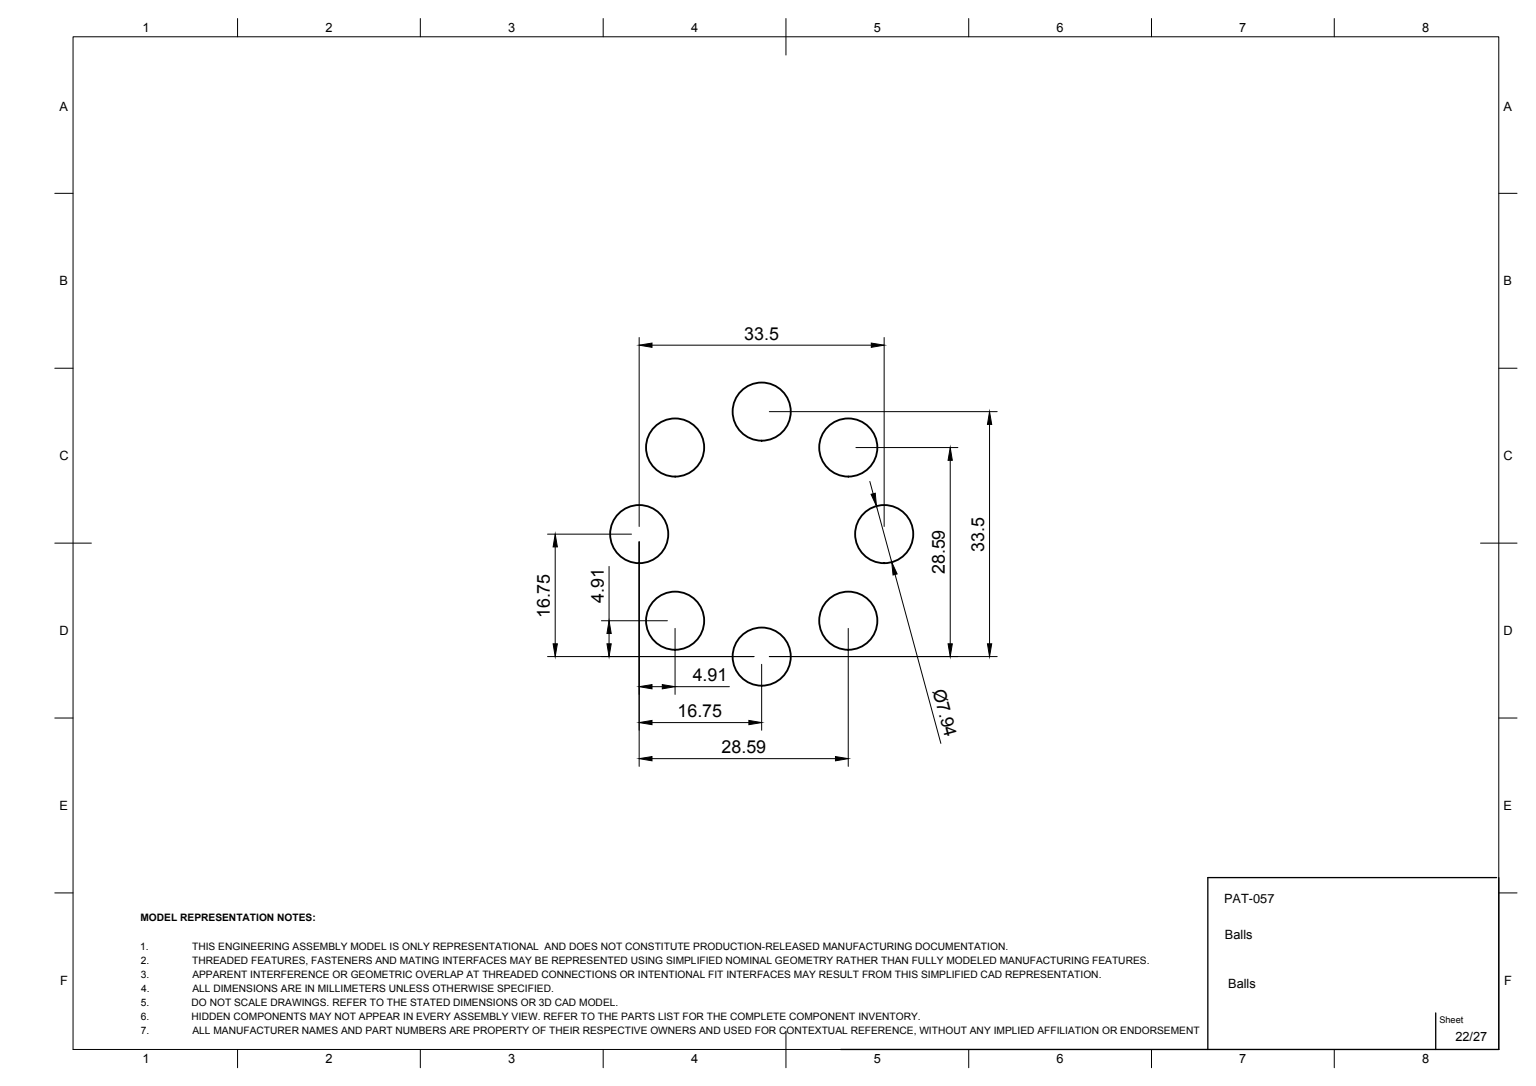
ISO-10303-21;
HEADER;
/* Generated by software containing ST-Developer
 * from STEP Tools, Inc. (www.steptools.com) 
 */

FILE_DESCRIPTION(
/* description */ ('Bearing-mounted hook block'),
/* implementation_level */ '2;1');

FILE_NAME(
/* name */ 'Balls.step',
/* time_stamp */ '2026-10-28T22:30:11-07:00',
/* author */ (''),
/* organization */ (''),
/* preprocessor_version */ 'ST-DEVELOPER v20.2',
/* originating_system */ 'Autodesk Translation Framework v15.17.0.0',
/* authorisation */ '');

FILE_SCHEMA (('AUTOMOTIVE_DESIGN { 1 0 10303 214 3 1 1 }'));
ENDSEC;

DATA;
#10=MECHANICAL_DESIGN_GEOMETRIC_PRESENTATION_REPRESENTATION('',(#339,#340,#341,#342,#343,#344,#345,#346),#7609);
#29=SPHERICAL_SURFACE('',#4545,0.3969);
#30=SPHERICAL_SURFACE('',#4547,0.3969);
#31=SPHERICAL_SURFACE('',#4549,0.3969);
#32=SPHERICAL_SURFACE('',#4551,0.3969);
#33=SPHERICAL_SURFACE('',#4553,0.3969);
#34=SPHERICAL_SURFACE('',#4555,0.3969);
#35=SPHERICAL_SURFACE('',#4557,0.3969);
#36=SPHERICAL_SURFACE('',#4559,0.3969);
#291=SHAPE_REPRESENTATION_RELATIONSHIP('SRR','None',#7740,#315);
#315=ADVANCED_BREP_SHAPE_REPRESENTATION('',(#369,#370,#371,#372,#373,#374,
#375,#376),#7600);
#339=STYLED_ITEM('',(#7931),#369);
#340=STYLED_ITEM('',(#7931),#370);
#341=STYLED_ITEM('',(#7931),#371);
#342=STYLED_ITEM('',(#7931),#372);
#343=STYLED_ITEM('',(#7931),#373);
#344=STYLED_ITEM('',(#7931),#374);
#345=STYLED_ITEM('',(#7931),#375);
#346=STYLED_ITEM('',(#7931),#376);
#369=MANIFOLD_SOLID_BREP('Body1',#3937);
#370=MANIFOLD_SOLID_BREP('Body2',#3938);
#371=MANIFOLD_SOLID_BREP('Body3',#3939);
#372=MANIFOLD_SOLID_BREP('Body4',#3940);
#373=MANIFOLD_SOLID_BREP('Body5',#3941);
#374=MANIFOLD_SOLID_BREP('Body6',#3942);
#375=MANIFOLD_SOLID_BREP('Body7',#3943);
#376=MANIFOLD_SOLID_BREP('Body8',#3944);
#1147=FACE_OUTER_BOUND('',#1440,.T.);
#1148=FACE_OUTER_BOUND('',#1441,.T.);
#1149=FACE_OUTER_BOUND('',#1442,.T.);
#1150=FACE_OUTER_BOUND('',#1443,.T.);
#1151=FACE_OUTER_BOUND('',#1444,.T.);
#1152=FACE_OUTER_BOUND('',#1445,.T.);
#1153=FACE_OUTER_BOUND('',#1446,.T.);
#1154=FACE_OUTER_BOUND('',#1447,.T.);
#1440=EDGE_LOOP('',(#3188,#3189));
#1441=EDGE_LOOP('',(#3190,#3191));
#1442=EDGE_LOOP('',(#3192,#3193));
#1443=EDGE_LOOP('',(#3194,#3195));
#1444=EDGE_LOOP('',(#3196,#3197));
#1445=EDGE_LOOP('',(#3198,#3199));
#1446=EDGE_LOOP('',(#3200,#3201));
#1447=EDGE_LOOP('',(#3202,#3203));
#1689=CIRCLE('',#4546,0.3969);
#1690=CIRCLE('',#4548,0.3969);
#1691=CIRCLE('',#4550,0.3969);
#1692=CIRCLE('',#4552,0.3969);
#1693=CIRCLE('',#4554,0.3969);
#1694=CIRCLE('',#4556,0.3969);
#1695=CIRCLE('',#4558,0.3969);
#1696=CIRCLE('',#4560,0.3969);
#1972=VERTEX_POINT('',#6771);
#1973=VERTEX_POINT('',#6772);
#1974=VERTEX_POINT('',#6775);
#1975=VERTEX_POINT('',#6776);
#1976=VERTEX_POINT('',#6779);
#1977=VERTEX_POINT('',#6780);
#1978=VERTEX_POINT('',#6783);
#1979=VERTEX_POINT('',#6784);
#1980=VERTEX_POINT('',#6787);
#1981=VERTEX_POINT('',#6788);
#1982=VERTEX_POINT('',#6791);
#1983=VERTEX_POINT('',#6792);
#1984=VERTEX_POINT('',#6795);
#1985=VERTEX_POINT('',#6796);
#1986=VERTEX_POINT('',#6799);
#1987=VERTEX_POINT('',#6800);
#2404=EDGE_CURVE('',#1972,#1973,#1689,.T.);
#2405=EDGE_CURVE('',#1974,#1975,#1690,.T.);
#2406=EDGE_CURVE('',#1976,#1977,#1691,.T.);
#2407=EDGE_CURVE('',#1978,#1979,#1692,.T.);
#2408=EDGE_CURVE('',#1980,#1981,#1693,.T.);
#2409=EDGE_CURVE('',#1982,#1983,#1694,.T.);
#2410=EDGE_CURVE('',#1984,#1985,#1695,.T.);
#2411=EDGE_CURVE('',#1986,#1987,#1696,.T.);
#3188=ORIENTED_EDGE('',*,*,#2404,.T.);
#3189=ORIENTED_EDGE('',*,*,#2404,.F.);
#3190=ORIENTED_EDGE('',*,*,#2405,.T.);
#3191=ORIENTED_EDGE('',*,*,#2405,.F.);
#3192=ORIENTED_EDGE('',*,*,#2406,.T.);
#3193=ORIENTED_EDGE('',*,*,#2406,.F.);
#3194=ORIENTED_EDGE('',*,*,#2407,.T.);
#3195=ORIENTED_EDGE('',*,*,#2407,.F.);
#3196=ORIENTED_EDGE('',*,*,#2408,.T.);
#3197=ORIENTED_EDGE('',*,*,#2408,.F.);
#3198=ORIENTED_EDGE('',*,*,#2409,.T.);
#3199=ORIENTED_EDGE('',*,*,#2409,.F.);
#3200=ORIENTED_EDGE('',*,*,#2410,.T.);
#3201=ORIENTED_EDGE('',*,*,#2410,.F.);
#3202=ORIENTED_EDGE('',*,*,#2411,.T.);
#3203=ORIENTED_EDGE('',*,*,#2411,.F.);
#3829=ADVANCED_FACE('',(#1147),#29,.T.);
#3830=ADVANCED_FACE('',(#1148),#30,.T.);
#3831=ADVANCED_FACE('',(#1149),#31,.T.);
#3832=ADVANCED_FACE('',(#1150),#32,.T.);
#3833=ADVANCED_FACE('',(#1151),#33,.T.);
#3834=ADVANCED_FACE('',(#1152),#34,.T.);
#3835=ADVANCED_FACE('',(#1153),#35,.T.);
#3836=ADVANCED_FACE('',(#1154),#36,.T.);
#3937=CLOSED_SHELL('',(#3829));
#3938=CLOSED_SHELL('',(#3830));
#3939=CLOSED_SHELL('',(#3831));
#3940=CLOSED_SHELL('',(#3832));
#3941=CLOSED_SHELL('',(#3833));
#3942=CLOSED_SHELL('',(#3834));
#3943=CLOSED_SHELL('',(#3835));
#3944=CLOSED_SHELL('',(#3836));
#4544=AXIS2_PLACEMENT_3D('',#6769,#5558,#5559);
#4545=AXIS2_PLACEMENT_3D('',#6770,#5560,#5561);
#4546=AXIS2_PLACEMENT_3D('',#6773,#5562,#5563);
#4547=AXIS2_PLACEMENT_3D('',#6774,#5564,#5565);
#4548=AXIS2_PLACEMENT_3D('',#6777,#5566,#5567);
#4549=AXIS2_PLACEMENT_3D('',#6778,#5568,#5569);
#4550=AXIS2_PLACEMENT_3D('',#6781,#5570,#5571);
#4551=AXIS2_PLACEMENT_3D('',#6782,#5572,#5573);
#4552=AXIS2_PLACEMENT_3D('',#6785,#5574,#5575);
#4553=AXIS2_PLACEMENT_3D('',#6786,#5576,#5577);
#4554=AXIS2_PLACEMENT_3D('',#6789,#5578,#5579);
#4555=AXIS2_PLACEMENT_3D('',#6790,#5580,#5581);
#4556=AXIS2_PLACEMENT_3D('',#6793,#5582,#5583);
#4557=AXIS2_PLACEMENT_3D('',#6794,#5584,#5585);
#4558=AXIS2_PLACEMENT_3D('',#6797,#5586,#5587);
#4559=AXIS2_PLACEMENT_3D('',#6798,#5588,#5589);
#4560=AXIS2_PLACEMENT_3D('',#6801,#5590,#5591);
#5558=DIRECTION('axis',(0.,0.,1.));
#5559=DIRECTION('refdir',(1.,0.,0.));
#5560=DIRECTION('center_axis',(0.,0.,1.));
#5561=DIRECTION('ref_axis',(1.,0.,0.));
#5562=DIRECTION('center_axis',(1.22464679914735E-16,-1.,0.));
#5563=DIRECTION('ref_axis',(-1.,-1.22464679914735E-16,0.));
#5564=DIRECTION('center_axis',(0.707106781186548,0.,0.707106781186548));
#5565=DIRECTION('ref_axis',(0.707106781186548,0.,-0.707106781186548));
#5566=DIRECTION('center_axis',(8.65956056235493E-17,-1.,-8.65956056235493E-17));
#5567=DIRECTION('ref_axis',(-0.707106781186548,-1.22464679914735E-16,0.707106781186548));
#5568=DIRECTION('center_axis',(1.,0.,0.));
#5569=DIRECTION('ref_axis',(6.12323399573677E-17,0.,-1.));
#5570=DIRECTION('center_axis',(7.49879891330929E-33,-1.,-1.22464679914735E-16));
#5571=DIRECTION('ref_axis',(-6.12323399573677E-17,-1.22464679914735E-16,
1.));
#5572=DIRECTION('center_axis',(0.707106781186548,0.,-0.707106781186548));
#5573=DIRECTION('ref_axis',(-0.707106781186548,0.,-0.707106781186548));
#5574=DIRECTION('center_axis',(-8.65956056235493E-17,-1.,-8.65956056235493E-17));
#5575=DIRECTION('ref_axis',(0.707106781186548,-1.22464679914735E-16,0.707106781186548));
#5576=DIRECTION('center_axis',(0.,0.,-1.));
#5577=DIRECTION('ref_axis',(-1.,0.,-1.22464679914735E-16));
#5578=DIRECTION('center_axis',(-1.22464679914735E-16,-1.,-1.49975978266186E-32));
#5579=DIRECTION('ref_axis',(1.,-1.22464679914735E-16,1.22464679914735E-16));
#5580=DIRECTION('center_axis',(-0.707106781186548,0.,-0.707106781186548));
#5581=DIRECTION('ref_axis',(-0.707106781186548,0.,0.707106781186548));
#5582=DIRECTION('center_axis',(-8.65956056235493E-17,-1.,8.65956056235493E-17));
#5583=DIRECTION('ref_axis',(0.707106781186548,-1.22464679914735E-16,-0.707106781186548));
#5584=DIRECTION('center_axis',(-1.,0.,0.));
#5585=DIRECTION('ref_axis',(-1.83697019872103E-16,0.,1.));
#5586=DIRECTION('center_axis',(-2.24963967399279E-32,-1.,1.22464679914735E-16));
#5587=DIRECTION('ref_axis',(1.83697019872103E-16,-1.22464679914735E-16,
-1.));
#5588=DIRECTION('center_axis',(-0.707106781186548,0.,0.707106781186548));
#5589=DIRECTION('ref_axis',(0.707106781186548,0.,0.707106781186548));
#5590=DIRECTION('center_axis',(8.65956056235493E-17,-1.,8.65956056235494E-17));
#5591=DIRECTION('ref_axis',(-0.707106781186548,-1.22464679914735E-16,-0.707106781186548));
#6769=CARTESIAN_POINT('',(0.,0.,0.));
#6770=CARTESIAN_POINT('Origin',(1.675,0.,0.));
#6771=CARTESIAN_POINT('',(1.675,-2.97627328869245E-33,0.3969));
#6772=CARTESIAN_POINT('',(1.675,-2.97627328869245E-33,-0.3969));
#6773=CARTESIAN_POINT('Origin',(1.675,0.,0.));
#6774=CARTESIAN_POINT('Origin',(1.18440385848747,0.,-1.18440385848747));
#6775=CARTESIAN_POINT('',(1.46505453994041,3.1867025333467E-33,-0.903753177034526));
#6776=CARTESIAN_POINT('',(0.903753177034527,-9.13924911073161E-33,-1.46505453994041));
#6777=CARTESIAN_POINT('Origin',(1.18440385848747,0.,-1.18440385848747));
#6778=CARTESIAN_POINT('Origin',(1.02564169428591E-16,0.,-1.675));
#6779=CARTESIAN_POINT('',(0.3969,-2.97627328869246E-33,-1.675));
#6780=CARTESIAN_POINT('',(-0.3969,-2.97627328869245E-33,-1.675));
#6781=CARTESIAN_POINT('Origin',(1.02564169428591E-16,0.,-1.675));
#6782=CARTESIAN_POINT('Origin',(-1.18440385848747,0.,-1.18440385848747));
#6783=CARTESIAN_POINT('',(-0.903753177034526,3.1867025333467E-33,-1.46505453994041));
#6784=CARTESIAN_POINT('',(-1.46505453994041,-9.13924911073161E-33,-0.903753177034527));
#6785=CARTESIAN_POINT('Origin',(-1.18440385848747,0.,-1.18440385848747));
#6786=CARTESIAN_POINT('Origin',(-1.675,0.,-2.05128338857182E-16));
#6787=CARTESIAN_POINT('',(-1.675,-2.97627328869246E-33,-0.3969));
#6788=CARTESIAN_POINT('',(-1.675,-2.97627328869245E-33,0.3969));
#6789=CARTESIAN_POINT('Origin',(-1.675,0.,-2.05128338857182E-16));
#6790=CARTESIAN_POINT('Origin',(-1.18440385848747,0.,1.18440385848747));
#6791=CARTESIAN_POINT('',(-1.46505453994041,6.26819044436628E-33,0.903753177034526));
#6792=CARTESIAN_POINT('',(-0.903753177034527,-1.22207370217512E-32,1.46505453994041));
#6793=CARTESIAN_POINT('Origin',(-1.18440385848747,0.,1.18440385848747));
#6794=CARTESIAN_POINT('Origin',(-3.07692508285772E-16,0.,1.675));
#6795=CARTESIAN_POINT('',(-0.3969,-2.97627328869246E-33,1.675));
#6796=CARTESIAN_POINT('',(0.396899999999999,-2.97627328869245E-33,1.675));
#6797=CARTESIAN_POINT('Origin',(-3.07692508285772E-16,0.,1.675));
#6798=CARTESIAN_POINT('Origin',(1.18440385848747,0.,1.18440385848747));
#6799=CARTESIAN_POINT('',(0.903753177034526,9.34967835538585E-33,1.46505453994041));
#6800=CARTESIAN_POINT('',(1.46505453994041,-1.53022249327708E-32,0.903753177034527));
#6801=CARTESIAN_POINT('Origin',(1.18440385848747,0.,1.18440385848747));
#7570=UNCERTAINTY_MEASURE_WITH_UNIT(LENGTH_MEASURE(0.001),#7610,
'DISTANCE_ACCURACY_VALUE',
'Maximum model space distance between geometric entities at asserted c
onnectivities');
#7579=UNCERTAINTY_MEASURE_WITH_UNIT(LENGTH_MEASURE(0.001),#7610,
'DISTANCE_ACCURACY_VALUE',
'Maximum model space distance between geometric entities at asserted c
onnectivities');
#7600=(
GEOMETRIC_REPRESENTATION_CONTEXT(3)
GLOBAL_UNCERTAINTY_ASSIGNED_CONTEXT((#7570))
GLOBAL_UNIT_ASSIGNED_CONTEXT((#7610,#7612,#7613))
REPRESENTATION_CONTEXT('','3D')
);
#7609=(
GEOMETRIC_REPRESENTATION_CONTEXT(3)
GLOBAL_UNCERTAINTY_ASSIGNED_CONTEXT((#7579))
GLOBAL_UNIT_ASSIGNED_CONTEXT((#7610,#7612,#7613))
REPRESENTATION_CONTEXT('','3D')
);
#7610=(
LENGTH_UNIT()
NAMED_UNIT(*)
SI_UNIT(.CENTI.,.METRE.)
);
#7612=(
NAMED_UNIT(*)
PLANE_ANGLE_UNIT()
SI_UNIT($,.RADIAN.)
);
#7613=(
NAMED_UNIT(*)
SI_UNIT($,.STERADIAN.)
SOLID_ANGLE_UNIT()
);
#7634=SHAPE_DEFINITION_REPRESENTATION(#7686,#7740);
#7686=PRODUCT_DEFINITION_SHAPE('',$,#7770);
#7740=SHAPE_REPRESENTATION('',(#4544),#7600);
#7749=PRODUCT_DEFINITION_CONTEXT('part definition',#7838,'design');
#7770=PRODUCT_DEFINITION('Balls','Balls',#7799,#7749);
#7799=PRODUCT_DEFINITION_FORMATION('',$,#7860);
#7838=APPLICATION_CONTEXT(
'Core Data for Automotive Mechanical Design Process');
#7839=PRODUCT_CONTEXT('part definition',#7838,'mechanical');
#7860=PRODUCT('Balls','Balls','Balls',(#7839));
#7925=COLOUR_RGB('Grey',0.48,0.52,0.57);
#7926=FILL_AREA_STYLE_COLOUR('',#7925);
#7927=FILL_AREA_STYLE('',(#7926));
#7928=SURFACE_STYLE_FILL_AREA(#7927);
#7929=SURFACE_SIDE_STYLE('',(#7928));
#7930=SURFACE_STYLE_USAGE(.BOTH.,#7929);
#7931=PRESENTATION_STYLE_ASSIGNMENT((#7930));
ENDSEC;
END-ISO-10303-21;
